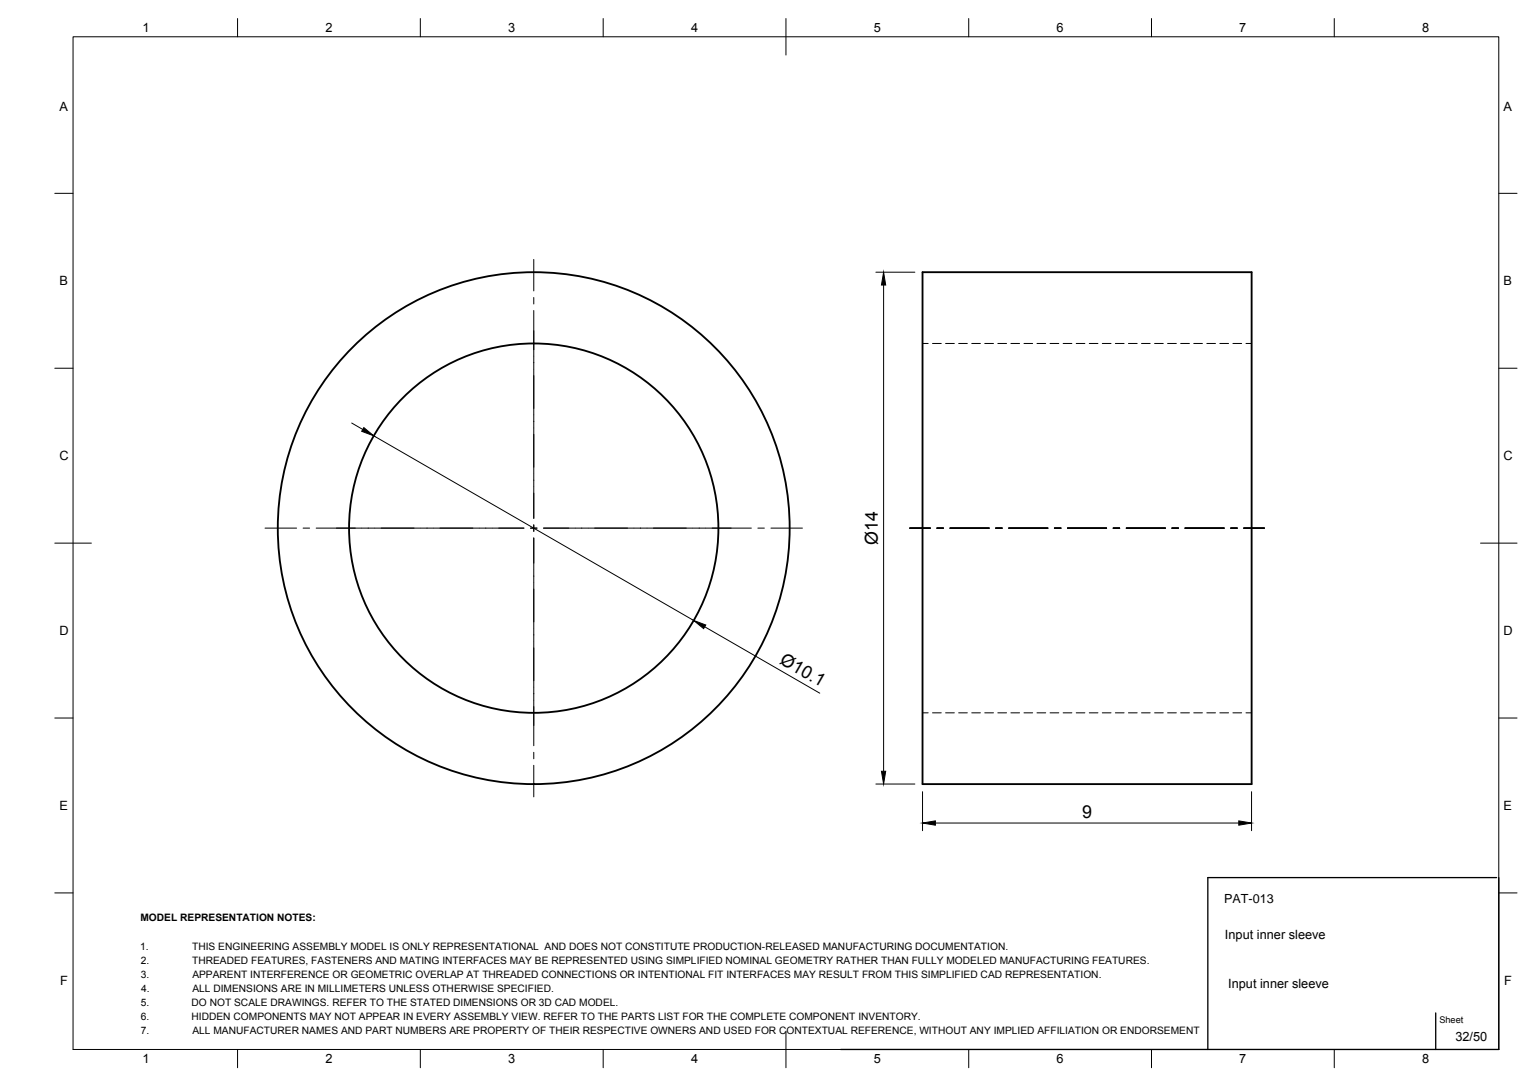
ISO-10303-21;
HEADER;
/* Generated by software containing ST-Developer
 * from STEP Tools, Inc. (www.steptools.com) 
 */

FILE_DESCRIPTION(
/* description */ ('Belt-driven linear axis on 2020 extrusion'),
/* implementation_level */ '2;1');

FILE_NAME(
/* name */ 'Input inner sleeve.step',
/* time_stamp */ '2026-10-28T03:26:09-07:00',
/* author */ (''),
/* organization */ (''),
/* preprocessor_version */ 'ST-DEVELOPER v20.2',
/* originating_system */ 'Autodesk Translation Framework v15.17.0.0',
/* authorisation */ '');

FILE_SCHEMA (('AUTOMOTIVE_DESIGN { 1 0 10303 214 3 1 1 }'));
ENDSEC;

DATA;
#10=MECHANICAL_DESIGN_GEOMETRIC_PRESENTATION_REPRESENTATION('',(#645),#20096);
#543=SHAPE_REPRESENTATION_RELATIONSHIP('SRR','None',#20341,#589);
#589=ADVANCED_BREP_SHAPE_REPRESENTATION('',(#700),#20072);
#645=STYLED_ITEM('',(#20636),#700);
#700=MANIFOLD_SOLID_BREP('Body1',#10959);
#836=FACE_BOUND('',#2378,.T.);
#837=FACE_BOUND('',#2380,.T.);
#1119=PLANE('',#12231);
#1120=PLANE('',#12232);
#1635=FACE_OUTER_BOUND('',#2375,.T.);
#1636=FACE_OUTER_BOUND('',#2376,.T.);
#1637=FACE_OUTER_BOUND('',#2377,.T.);
#1638=FACE_OUTER_BOUND('',#2379,.T.);
#2375=EDGE_LOOP('',(#9013,#9014,#9015,#9016));
#2376=EDGE_LOOP('',(#9017,#9018,#9019,#9020));
#2377=EDGE_LOOP('',(#9021));
#2378=EDGE_LOOP('',(#9022));
#2379=EDGE_LOOP('',(#9023));
#2380=EDGE_LOOP('',(#9024));
#3212=LINE('',#18469,#4069);
#3213=LINE('',#18475,#4070);
#4069=VECTOR('',#14806,0.505);
#4070=VECTOR('',#14813,0.7);
#4692=CIRCLE('',#12226,0.505);
#4693=CIRCLE('',#12227,0.505);
#4694=CIRCLE('',#12229,0.7);
#4695=CIRCLE('',#12230,0.7);
#5487=VERTEX_POINT('',#18466);
#5488=VERTEX_POINT('',#18468);
#5489=VERTEX_POINT('',#18472);
#5490=VERTEX_POINT('',#18474);
#6721=EDGE_CURVE('',#5487,#5487,#4692,.T.);
#6722=EDGE_CURVE('',#5487,#5488,#3212,.T.);
#6723=EDGE_CURVE('',#5488,#5488,#4693,.T.);
#6724=EDGE_CURVE('',#5489,#5489,#4694,.T.);
#6725=EDGE_CURVE('',#5489,#5490,#3213,.T.);
#6726=EDGE_CURVE('',#5490,#5490,#4695,.T.);
#9013=ORIENTED_EDGE('',*,*,#6721,.F.);
#9014=ORIENTED_EDGE('',*,*,#6722,.T.);
#9015=ORIENTED_EDGE('',*,*,#6723,.T.);
#9016=ORIENTED_EDGE('',*,*,#6722,.F.);
#9017=ORIENTED_EDGE('',*,*,#6724,.F.);
#9018=ORIENTED_EDGE('',*,*,#6725,.T.);
#9019=ORIENTED_EDGE('',*,*,#6726,.T.);
#9020=ORIENTED_EDGE('',*,*,#6725,.F.);
#9021=ORIENTED_EDGE('',*,*,#6724,.T.);
#9022=ORIENTED_EDGE('',*,*,#6721,.T.);
#9023=ORIENTED_EDGE('',*,*,#6726,.F.);
#9024=ORIENTED_EDGE('',*,*,#6723,.F.);
#10207=CYLINDRICAL_SURFACE('',#12225,0.505);
#10208=CYLINDRICAL_SURFACE('',#12228,0.7);
#10686=ADVANCED_FACE('',(#1635),#10207,.F.);
#10687=ADVANCED_FACE('',(#1636),#10208,.T.);
#10688=ADVANCED_FACE('',(#1637,#836),#1119,.T.);
#10689=ADVANCED_FACE('',(#1638,#837),#1120,.F.);
#10959=CLOSED_SHELL('',(#10686,#10687,#10688,#10689));
#12224=AXIS2_PLACEMENT_3D('',#18464,#14800,#14801);
#12225=AXIS2_PLACEMENT_3D('',#18465,#14802,#14803);
#12226=AXIS2_PLACEMENT_3D('',#18467,#14804,#14805);
#12227=AXIS2_PLACEMENT_3D('',#18470,#14807,#14808);
#12228=AXIS2_PLACEMENT_3D('',#18471,#14809,#14810);
#12229=AXIS2_PLACEMENT_3D('',#18473,#14811,#14812);
#12230=AXIS2_PLACEMENT_3D('',#18476,#14814,#14815);
#12231=AXIS2_PLACEMENT_3D('',#18477,#14816,#14817);
#12232=AXIS2_PLACEMENT_3D('',#18478,#14818,#14819);
#14800=DIRECTION('axis',(0.,0.,1.));
#14801=DIRECTION('refdir',(1.,0.,0.));
#14802=DIRECTION('center_axis',(0.,1.,0.));
#14803=DIRECTION('ref_axis',(1.,0.,0.));
#14804=DIRECTION('center_axis',(0.,-1.,0.));
#14805=DIRECTION('ref_axis',(1.,0.,0.));
#14806=DIRECTION('',(0.,-1.,0.));
#14807=DIRECTION('center_axis',(0.,-1.,0.));
#14808=DIRECTION('ref_axis',(1.,0.,0.));
#14809=DIRECTION('center_axis',(0.,1.,0.));
#14810=DIRECTION('ref_axis',(1.,0.,0.));
#14811=DIRECTION('center_axis',(0.,1.,0.));
#14812=DIRECTION('ref_axis',(1.,0.,0.));
#14813=DIRECTION('',(0.,-1.,0.));
#14814=DIRECTION('center_axis',(0.,1.,0.));
#14815=DIRECTION('ref_axis',(1.,0.,0.));
#14816=DIRECTION('center_axis',(0.,1.,0.));
#14817=DIRECTION('ref_axis',(1.,0.,0.));
#14818=DIRECTION('center_axis',(0.,1.,0.));
#14819=DIRECTION('ref_axis',(1.,0.,0.));
#18464=CARTESIAN_POINT('',(0.,0.,0.));
#18465=CARTESIAN_POINT('Origin',(0.,-0.45,7.));
#18466=CARTESIAN_POINT('',(-0.505,0.45,7.));
#18467=CARTESIAN_POINT('Origin',(0.,0.45,7.));
#18468=CARTESIAN_POINT('',(-0.505,-0.45,7.));
#18469=CARTESIAN_POINT('',(-0.505,-0.45,7.));
#18470=CARTESIAN_POINT('Origin',(0.,-0.45,7.));
#18471=CARTESIAN_POINT('Origin',(0.,-0.45,7.));
#18472=CARTESIAN_POINT('',(-0.7,0.45,7.));
#18473=CARTESIAN_POINT('Origin',(0.,0.45,7.));
#18474=CARTESIAN_POINT('',(-0.7,-0.45,7.));
#18475=CARTESIAN_POINT('',(-0.7,-0.45,7.));
#18476=CARTESIAN_POINT('Origin',(0.,-0.45,7.));
#18477=CARTESIAN_POINT('Origin',(0.,0.45,7.));
#18478=CARTESIAN_POINT('Origin',(0.,-0.45,7.));
#20018=UNCERTAINTY_MEASURE_WITH_UNIT(LENGTH_MEASURE(0.001),#20097,
'DISTANCE_ACCURACY_VALUE',
'Maximum model space distance between geometric entities at asserted c
onnectivities');
#20042=UNCERTAINTY_MEASURE_WITH_UNIT(LENGTH_MEASURE(0.001),#20097,
'DISTANCE_ACCURACY_VALUE',
'Maximum model space distance between geometric entities at asserted c
onnectivities');
#20072=(
GEOMETRIC_REPRESENTATION_CONTEXT(3)
GLOBAL_UNCERTAINTY_ASSIGNED_CONTEXT((#20018))
GLOBAL_UNIT_ASSIGNED_CONTEXT((#20097,#20099,#20100))
REPRESENTATION_CONTEXT('','3D')
);
#20096=(
GEOMETRIC_REPRESENTATION_CONTEXT(3)
GLOBAL_UNCERTAINTY_ASSIGNED_CONTEXT((#20042))
GLOBAL_UNIT_ASSIGNED_CONTEXT((#20097,#20099,#20100))
REPRESENTATION_CONTEXT('','3D')
);
#20097=(
LENGTH_UNIT()
NAMED_UNIT(*)
SI_UNIT(.CENTI.,.METRE.)
);
#20099=(
NAMED_UNIT(*)
PLANE_ANGLE_UNIT()
SI_UNIT($,.RADIAN.)
);
#20100=(
NAMED_UNIT(*)
SI_UNIT($,.STERADIAN.)
SOLID_ANGLE_UNIT()
);
#20130=SHAPE_DEFINITION_REPRESENTATION(#20188,#20341);
#20188=PRODUCT_DEFINITION_SHAPE('',$,#20395);
#20341=SHAPE_REPRESENTATION('',(#12224),#20072);
#20365=PRODUCT_DEFINITION_CONTEXT('part definition',#20526,'design');
#20395=PRODUCT_DEFINITION('Input inner sleeve','Input inner sleeve',#20448,
#20365);
#20448=PRODUCT_DEFINITION_FORMATION('',$,#20557);
#20526=APPLICATION_CONTEXT(
'Core Data for Automotive Mechanical Design Process');
#20527=PRODUCT_CONTEXT('part definition',#20526,'mechanical');
#20557=PRODUCT('Input inner sleeve','Input inner sleeve',
'Input inner sleeve',(#20527));
#20630=COLOUR_RGB('Light Blue',0.38,0.62,0.78);
#20631=FILL_AREA_STYLE_COLOUR('',#20630);
#20632=FILL_AREA_STYLE('',(#20631));
#20633=SURFACE_STYLE_FILL_AREA(#20632);
#20634=SURFACE_SIDE_STYLE('',(#20633));
#20635=SURFACE_STYLE_USAGE(.BOTH.,#20634);
#20636=PRESENTATION_STYLE_ASSIGNMENT((#20635));
ENDSEC;
END-ISO-10303-21;
